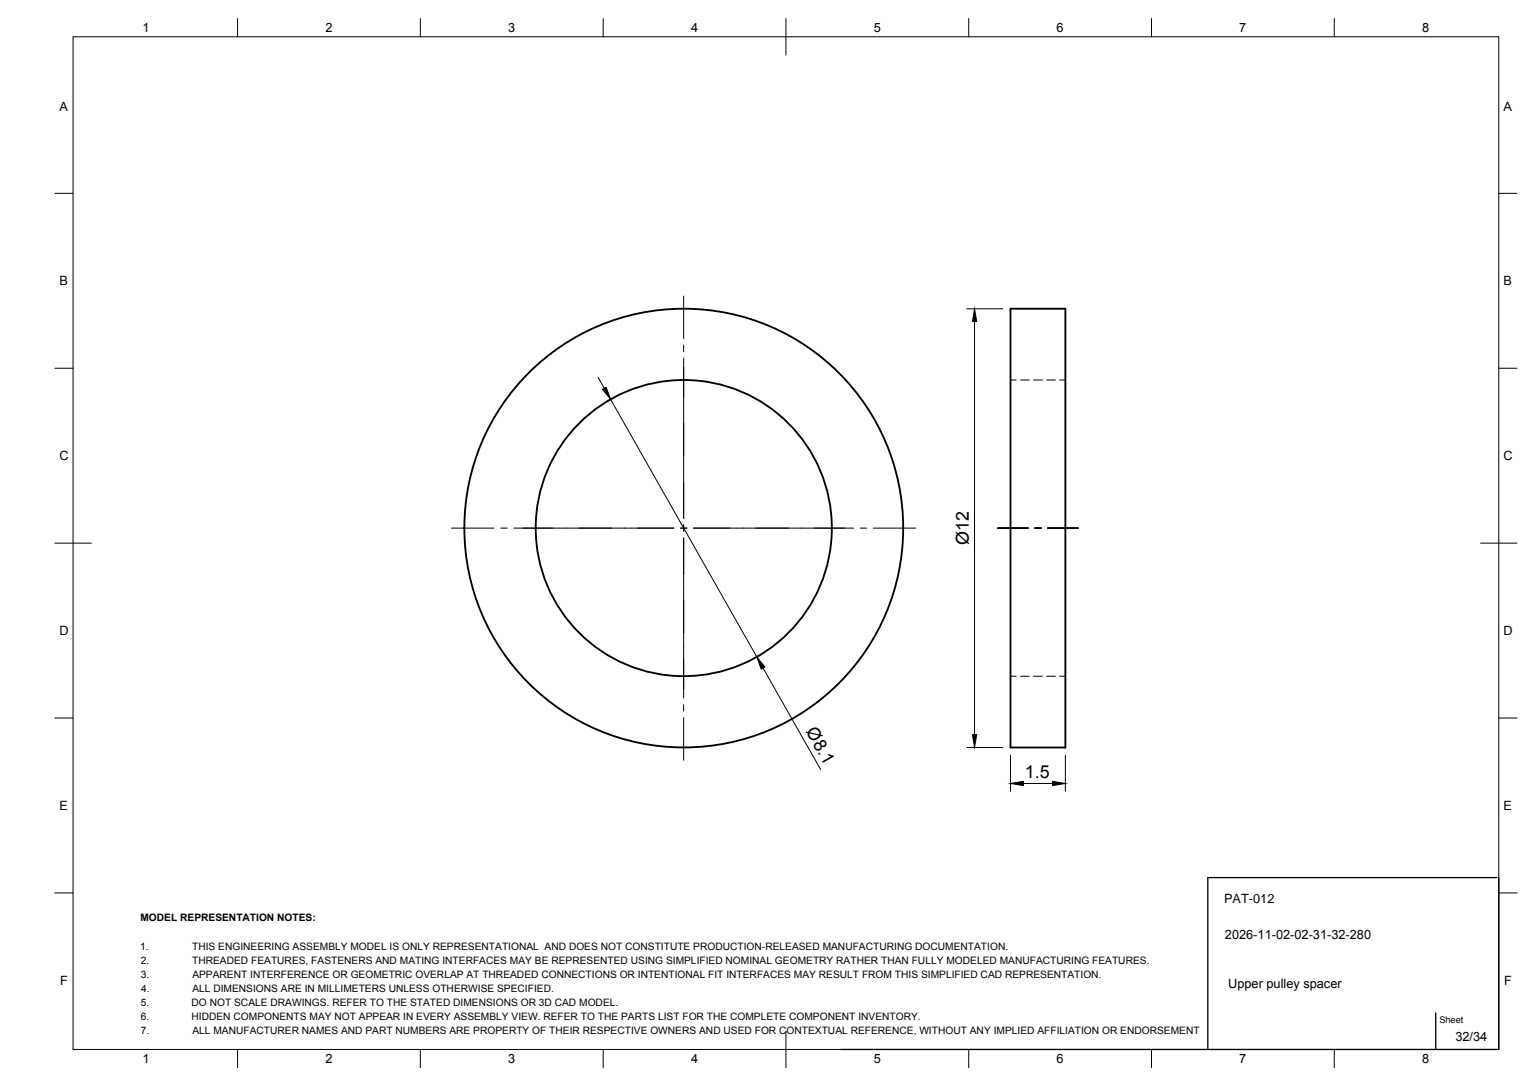
ISO-10303-21;
HEADER;
/* Generated by software containing ST-Developer
 * from STEP Tools, Inc. (www.steptools.com) 
 */

FILE_DESCRIPTION(
/* description */ ('Belt tensioner idler arm'),
/* implementation_level */ '2;1');

FILE_NAME(
/* name */ 'Upper pulley spacer.step',
/* time_stamp */ '2026-10-28T03:22:15-07:00',
/* author */ (''),
/* organization */ (''),
/* preprocessor_version */ 'ST-DEVELOPER v20.2',
/* originating_system */ 'Autodesk Translation Framework v15.17.0.0',
/* authorisation */ '');

FILE_SCHEMA (('AUTOMOTIVE_DESIGN { 1 0 10303 214 3 1 1 }'));
ENDSEC;

DATA;
#10=MECHANICAL_DESIGN_GEOMETRIC_PRESENTATION_REPRESENTATION('',(#482),#12779);
#406=SHAPE_REPRESENTATION_RELATIONSHIP('SRR','None',#12955,#440);
#440=ADVANCED_BREP_SHAPE_REPRESENTATION('',(#521),#12772);
#482=STYLED_ITEM('',(#13170),#521);
#521=MANIFOLD_SOLID_BREP('Body1',#6219);
#646=FACE_BOUND('',#1599,.T.);
#647=FACE_BOUND('',#1601,.T.);
#804=PLANE('',#7197);
#805=PLANE('',#7198);
#1110=FACE_OUTER_BOUND('',#1596,.T.);
#1111=FACE_OUTER_BOUND('',#1597,.T.);
#1112=FACE_OUTER_BOUND('',#1598,.T.);
#1113=FACE_OUTER_BOUND('',#1600,.T.);
#1596=EDGE_LOOP('',(#5200,#5201,#5202,#5203));
#1597=EDGE_LOOP('',(#5204,#5205,#5206,#5207));
#1598=EDGE_LOOP('',(#5208));
#1599=EDGE_LOOP('',(#5209));
#1600=EDGE_LOOP('',(#5210));
#1601=EDGE_LOOP('',(#5211));
#1957=LINE('',#11907,#2306);
#1958=LINE('',#11913,#2307);
#2306=VECTOR('',#8865,0.404999999999999);
#2307=VECTOR('',#8872,0.6);
#2659=CIRCLE('',#7192,0.404999999999999);
#2660=CIRCLE('',#7193,0.404999999999999);
#2661=CIRCLE('',#7195,0.6);
#2662=CIRCLE('',#7196,0.6);
#3142=VERTEX_POINT('',#11904);
#3143=VERTEX_POINT('',#11906);
#3144=VERTEX_POINT('',#11910);
#3145=VERTEX_POINT('',#11912);
#3855=EDGE_CURVE('',#3142,#3142,#2659,.T.);
#3856=EDGE_CURVE('',#3142,#3143,#1957,.T.);
#3857=EDGE_CURVE('',#3143,#3143,#2660,.T.);
#3858=EDGE_CURVE('',#3144,#3144,#2661,.T.);
#3859=EDGE_CURVE('',#3144,#3145,#1958,.T.);
#3860=EDGE_CURVE('',#3145,#3145,#2662,.T.);
#5200=ORIENTED_EDGE('',*,*,#3855,.F.);
#5201=ORIENTED_EDGE('',*,*,#3856,.T.);
#5202=ORIENTED_EDGE('',*,*,#3857,.T.);
#5203=ORIENTED_EDGE('',*,*,#3856,.F.);
#5204=ORIENTED_EDGE('',*,*,#3858,.F.);
#5205=ORIENTED_EDGE('',*,*,#3859,.T.);
#5206=ORIENTED_EDGE('',*,*,#3860,.T.);
#5207=ORIENTED_EDGE('',*,*,#3859,.F.);
#5208=ORIENTED_EDGE('',*,*,#3858,.T.);
#5209=ORIENTED_EDGE('',*,*,#3855,.T.);
#5210=ORIENTED_EDGE('',*,*,#3860,.F.);
#5211=ORIENTED_EDGE('',*,*,#3857,.F.);
#5757=CYLINDRICAL_SURFACE('',#7191,0.404999999999999);
#5758=CYLINDRICAL_SURFACE('',#7194,0.6);
#6087=ADVANCED_FACE('',(#1110),#5757,.F.);
#6088=ADVANCED_FACE('',(#1111),#5758,.T.);
#6089=ADVANCED_FACE('',(#1112,#646),#804,.T.);
#6090=ADVANCED_FACE('',(#1113,#647),#805,.F.);
#6219=CLOSED_SHELL('',(#6087,#6088,#6089,#6090));
#7190=AXIS2_PLACEMENT_3D('',#11902,#8859,#8860);
#7191=AXIS2_PLACEMENT_3D('',#11903,#8861,#8862);
#7192=AXIS2_PLACEMENT_3D('',#11905,#8863,#8864);
#7193=AXIS2_PLACEMENT_3D('',#11908,#8866,#8867);
#7194=AXIS2_PLACEMENT_3D('',#11909,#8868,#8869);
#7195=AXIS2_PLACEMENT_3D('',#11911,#8870,#8871);
#7196=AXIS2_PLACEMENT_3D('',#11914,#8873,#8874);
#7197=AXIS2_PLACEMENT_3D('',#11915,#8875,#8876);
#7198=AXIS2_PLACEMENT_3D('',#11916,#8877,#8878);
#8859=DIRECTION('axis',(0.,0.,1.));
#8860=DIRECTION('refdir',(1.,0.,0.));
#8861=DIRECTION('center_axis',(0.,0.,1.));
#8862=DIRECTION('ref_axis',(1.,0.,0.));
#8863=DIRECTION('center_axis',(0.,0.,-1.));
#8864=DIRECTION('ref_axis',(1.,0.,0.));
#8865=DIRECTION('',(0.,0.,-1.));
#8866=DIRECTION('center_axis',(0.,0.,-1.));
#8867=DIRECTION('ref_axis',(1.,0.,0.));
#8868=DIRECTION('center_axis',(0.,0.,1.));
#8869=DIRECTION('ref_axis',(1.,0.,0.));
#8870=DIRECTION('center_axis',(0.,0.,1.));
#8871=DIRECTION('ref_axis',(1.,0.,0.));
#8872=DIRECTION('',(0.,0.,-1.));
#8873=DIRECTION('center_axis',(0.,0.,1.));
#8874=DIRECTION('ref_axis',(1.,0.,0.));
#8875=DIRECTION('center_axis',(0.,0.,1.));
#8876=DIRECTION('ref_axis',(1.,0.,0.));
#8877=DIRECTION('center_axis',(0.,0.,1.));
#8878=DIRECTION('ref_axis',(1.,0.,0.));
#11902=CARTESIAN_POINT('',(0.,0.,0.));
#11903=CARTESIAN_POINT('Origin',(9.,0.,8.85));
#11904=CARTESIAN_POINT('',(8.595,-4.95981953654677E-17,9.));
#11905=CARTESIAN_POINT('Origin',(9.,0.,9.));
#11906=CARTESIAN_POINT('',(8.595,-4.95981953654677E-17,8.85));
#11907=CARTESIAN_POINT('',(8.595,-4.95981953654677E-17,8.85));
#11908=CARTESIAN_POINT('Origin',(9.,0.,8.85));
#11909=CARTESIAN_POINT('Origin',(9.,0.,8.85));
#11910=CARTESIAN_POINT('',(8.4,-7.34788079488412E-17,9.));
#11911=CARTESIAN_POINT('Origin',(9.,0.,9.));
#11912=CARTESIAN_POINT('',(8.4,-7.34788079488412E-17,8.85));
#11913=CARTESIAN_POINT('',(8.4,-7.34788079488412E-17,8.85));
#11914=CARTESIAN_POINT('Origin',(9.,0.,8.85));
#11915=CARTESIAN_POINT('Origin',(9.,0.,9.));
#11916=CARTESIAN_POINT('Origin',(9.,0.,8.85));
#12732=UNCERTAINTY_MEASURE_WITH_UNIT(LENGTH_MEASURE(0.001),#12780,
'DISTANCE_ACCURACY_VALUE',
'Maximum model space distance between geometric entities at asserted c
onnectivities');
#12739=UNCERTAINTY_MEASURE_WITH_UNIT(LENGTH_MEASURE(0.001),#12780,
'DISTANCE_ACCURACY_VALUE',
'Maximum model space distance between geometric entities at asserted c
onnectivities');
#12772=(
GEOMETRIC_REPRESENTATION_CONTEXT(3)
GLOBAL_UNCERTAINTY_ASSIGNED_CONTEXT((#12732))
GLOBAL_UNIT_ASSIGNED_CONTEXT((#12780,#12782,#12783))
REPRESENTATION_CONTEXT('','3D')
);
#12779=(
GEOMETRIC_REPRESENTATION_CONTEXT(3)
GLOBAL_UNCERTAINTY_ASSIGNED_CONTEXT((#12739))
GLOBAL_UNIT_ASSIGNED_CONTEXT((#12780,#12782,#12783))
REPRESENTATION_CONTEXT('','3D')
);
#12780=(
LENGTH_UNIT()
NAMED_UNIT(*)
SI_UNIT(.CENTI.,.METRE.)
);
#12782=(
NAMED_UNIT(*)
PLANE_ANGLE_UNIT()
SI_UNIT($,.RADIAN.)
);
#12783=(
NAMED_UNIT(*)
SI_UNIT($,.STERADIAN.)
SOLID_ANGLE_UNIT()
);
#12816=SHAPE_DEFINITION_REPRESENTATION(#12884,#12955);
#12884=PRODUCT_DEFINITION_SHAPE('',$,#12995);
#12955=SHAPE_REPRESENTATION('',(#7190),#12772);
#12962=PRODUCT_DEFINITION_CONTEXT('part definition',#13081,'design');
#12995=PRODUCT_DEFINITION('Upper pulley spacer','Upper pulley spacer',#13034,
#12962);
#13034=PRODUCT_DEFINITION_FORMATION('',$,#13115);
#13081=APPLICATION_CONTEXT(
'Core Data for Automotive Mechanical Design Process');
#13082=PRODUCT_CONTEXT('part definition',#13081,'mechanical');
#13115=PRODUCT('Upper pulley spacer','Upper pulley spacer',
'Upper pulley spacer',(#13082));
#13164=COLOUR_RGB('Light Blue',0.38,0.62,0.78);
#13165=FILL_AREA_STYLE_COLOUR('',#13164);
#13166=FILL_AREA_STYLE('',(#13165));
#13167=SURFACE_STYLE_FILL_AREA(#13166);
#13168=SURFACE_SIDE_STYLE('',(#13167));
#13169=SURFACE_STYLE_USAGE(.BOTH.,#13168);
#13170=PRESENTATION_STYLE_ASSIGNMENT((#13169));
ENDSEC;
END-ISO-10303-21;
